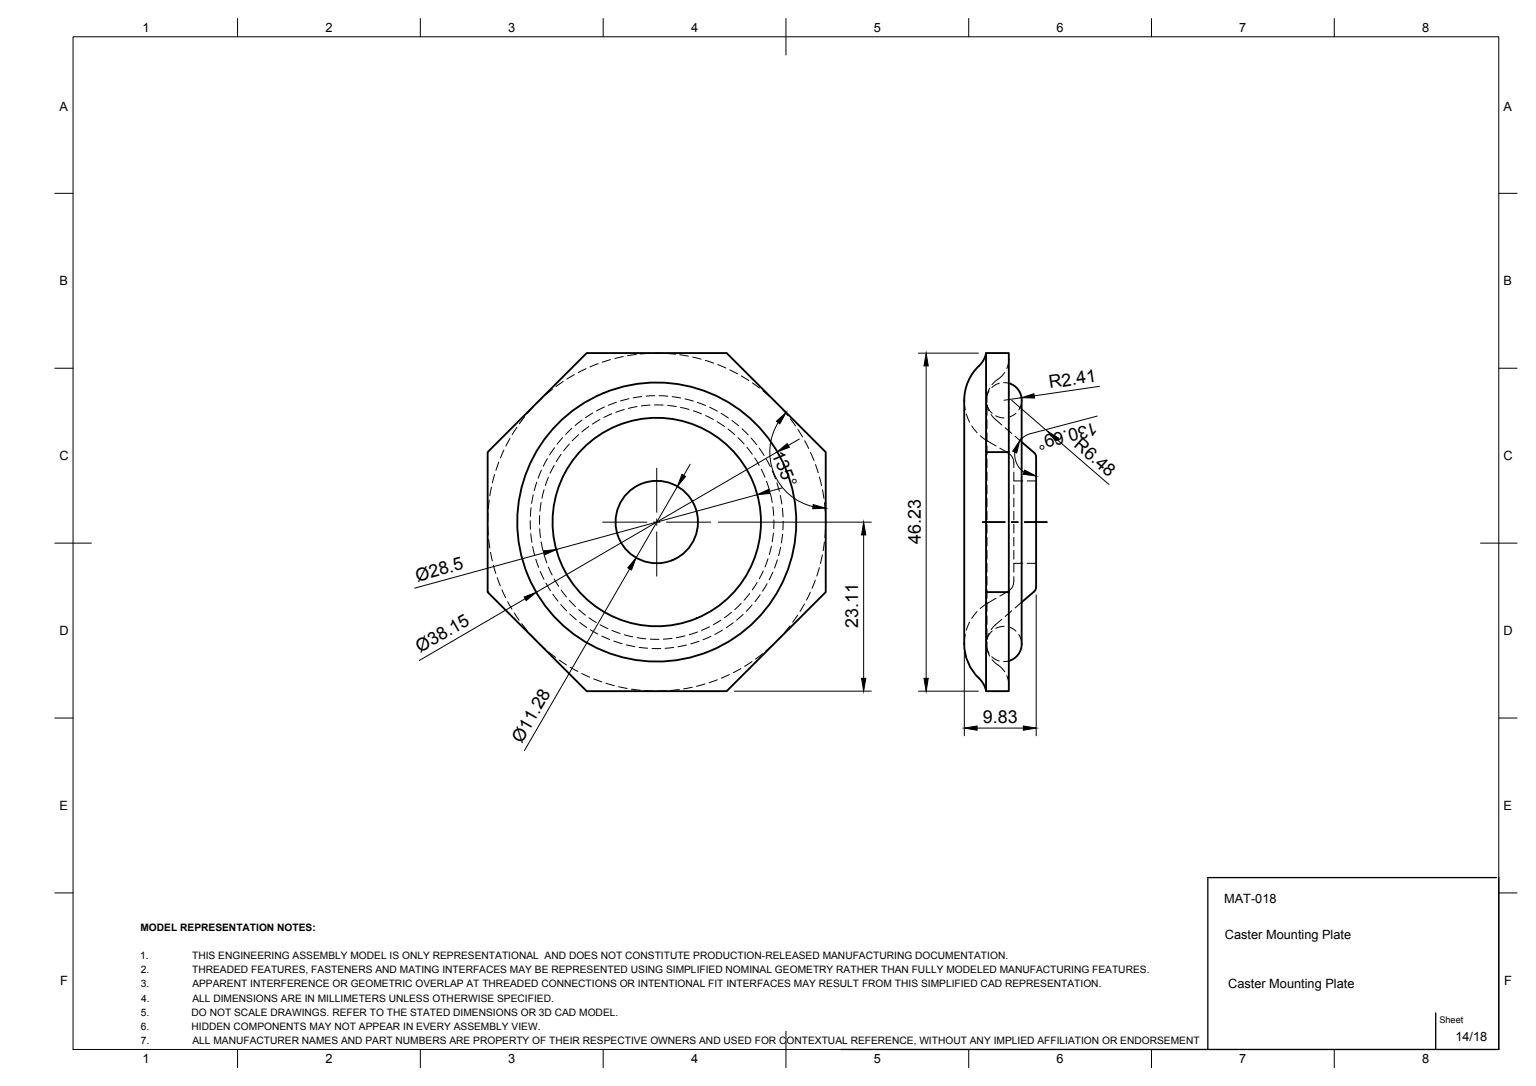
ISO-10303-21;
HEADER;
/* Generated by software containing ST-Developer
 * from STEP Tools, Inc. (www.steptools.com) 
 */

FILE_DESCRIPTION(
/* description */ ('STEP AP214'),
/* implementation_level */ '2;1');

FILE_NAME(
/* name */ 'Caster Mounting Plate.step',
/* time_stamp */ '2026-11-14T06:16:09-08:00',
/* author */ (''),
/* organization */ (''),
/* preprocessor_version */ 'ST-DEVELOPER v20.2',
/* originating_system */ 'Autodesk Translation Framework v15.17.0.0',
/* authorisation */ '');

FILE_SCHEMA (('AUTOMOTIVE_DESIGN { 1 0 10303 214 3 1 1 }'));
ENDSEC;

DATA;
#10=MECHANICAL_DESIGN_GEOMETRIC_PRESENTATION_REPRESENTATION('',(#358),#18006);
#141=CONICAL_SURFACE('',#10700,9.49667180024818,0.710179331162308);
#142=CONICAL_SURFACE('',#10715,11.0475234888716,0.521857699344453);
#252=TOROIDAL_SURFACE('',#10684,16.6624,2.413127);
#253=TOROIDAL_SURFACE('',#10688,16.6624,3.429);
#254=TOROIDAL_SURFACE('',#10695,8.89,0.8001);
#255=TOROIDAL_SURFACE('',#10701,16.6624,3.429);
#256=TOROIDAL_SURFACE('',#10704,22.296392545256,3.302);
#257=TOROIDAL_SURFACE('',#10707,23.7562339422346,3.302);
#258=TOROIDAL_SURFACE('',#10711,16.6624,6.477);
#259=TOROIDAL_SURFACE('',#10718,8.0899,1.6002);
#326=SHAPE_REPRESENTATION_RELATIONSHIP('SRR','None',#18084,#342);
#342=ADVANCED_BREP_SHAPE_REPRESENTATION('',(#374),#18001);
#358=STYLED_ITEM('',(#18172),#374);
#374=MANIFOLD_SOLID_BREP('Body1',#9567);
#482=FACE_BOUND('',#2048,.T.);
#483=FACE_BOUND('',#2050,.T.);
#484=FACE_BOUND('',#2052,.T.);
#485=FACE_BOUND('',#2054,.T.);
#813=PLANE('',#10721);
#814=PLANE('',#10722);
#815=PLANE('',#10723);
#816=PLANE('',#10724);
#817=PLANE('',#10725);
#818=PLANE('',#10726);
#819=PLANE('',#10727);
#820=PLANE('',#10728);
#821=PLANE('',#10729);
#822=PLANE('',#10730);
#823=PLANE('',#10731);
#824=PLANE('',#10732);
#1349=FACE_OUTER_BOUND('',#2028,.T.);
#1350=FACE_OUTER_BOUND('',#2029,.T.);
#1351=FACE_OUTER_BOUND('',#2030,.T.);
#1352=FACE_OUTER_BOUND('',#2031,.T.);
#1353=FACE_OUTER_BOUND('',#2032,.T.);
#1354=FACE_OUTER_BOUND('',#2033,.T.);
#1355=FACE_OUTER_BOUND('',#2034,.T.);
#1356=FACE_OUTER_BOUND('',#2035,.T.);
#1357=FACE_OUTER_BOUND('',#2036,.T.);
#1358=FACE_OUTER_BOUND('',#2037,.T.);
#1359=FACE_OUTER_BOUND('',#2038,.T.);
#1360=FACE_OUTER_BOUND('',#2039,.T.);
#1361=FACE_OUTER_BOUND('',#2040,.T.);
#1362=FACE_OUTER_BOUND('',#2041,.T.);
#1363=FACE_OUTER_BOUND('',#2042,.T.);
#1364=FACE_OUTER_BOUND('',#2043,.T.);
#1365=FACE_OUTER_BOUND('',#2044,.T.);
#1366=FACE_OUTER_BOUND('',#2045,.T.);
#1367=FACE_OUTER_BOUND('',#2046,.T.);
#1368=FACE_OUTER_BOUND('',#2047,.T.);
#1369=FACE_OUTER_BOUND('',#2049,.T.);
#1370=FACE_OUTER_BOUND('',#2051,.T.);
#1371=FACE_OUTER_BOUND('',#2053,.T.);
#2028=EDGE_LOOP('',(#8544,#8545,#8546,#8547));
#2029=EDGE_LOOP('',(#8548,#8549,#8550,#8551,#8552));
#2030=EDGE_LOOP('',(#8553,#8554,#8555,#8556));
#2031=EDGE_LOOP('',(#8557,#8558,#8559,#8560,#8561));
#2032=EDGE_LOOP('',(#8562,#8563,#8564,#8565,#8566,#8567));
#2033=EDGE_LOOP('',(#8568,#8569,#8570,#8571));
#2034=EDGE_LOOP('',(#8572,#8573,#8574,#8575));
#2035=EDGE_LOOP('',(#8576,#8577,#8578,#8579));
#2036=EDGE_LOOP('',(#8580,#8581,#8582,#8583,#8584));
#2037=EDGE_LOOP('',(#8585,#8586,#8587,#8588,#8589,#8590));
#2038=EDGE_LOOP('',(#8591,#8592,#8593,#8594,#8595));
#2039=EDGE_LOOP('',(#8596,#8597,#8598,#8599));
#2040=EDGE_LOOP('',(#8600,#8601,#8602,#8603));
#2041=EDGE_LOOP('',(#8604,#8605,#8606,#8607));
#2042=EDGE_LOOP('',(#8608,#8609,#8610,#8611));
#2043=EDGE_LOOP('',(#8612,#8613,#8614,#8615));
#2044=EDGE_LOOP('',(#8616,#8617,#8618,#8619));
#2045=EDGE_LOOP('',(#8620,#8621,#8622,#8623));
#2046=EDGE_LOOP('',(#8624,#8625,#8626,#8627));
#2047=EDGE_LOOP('',(#8628,#8629,#8630,#8631,#8632,#8633,#8634,#8635));
#2048=EDGE_LOOP('',(#8636));
#2049=EDGE_LOOP('',(#8637,#8638,#8639,#8640,#8641,#8642,#8643,#8644));
#2050=EDGE_LOOP('',(#8645));
#2051=EDGE_LOOP('',(#8646));
#2052=EDGE_LOOP('',(#8647));
#2053=EDGE_LOOP('',(#8648));
#2054=EDGE_LOOP('',(#8649));
#2792=LINE('',#17674,#3516);
#2793=LINE('',#17685,#3517);
#2794=LINE('',#17710,#3518);
#2795=LINE('',#17719,#3519);
#2796=LINE('',#17721,#3520);
#2797=LINE('',#17723,#3521);
#2798=LINE('',#17724,#3522);
#2799=LINE('',#17727,#3523);
#2800=LINE('',#17729,#3524);
#2801=LINE('',#17730,#3525);
#2802=LINE('',#17733,#3526);
#2803=LINE('',#17735,#3527);
#2804=LINE('',#17736,#3528);
#2805=LINE('',#17739,#3529);
#2806=LINE('',#17741,#3530);
#2807=LINE('',#17742,#3531);
#2808=LINE('',#17745,#3532);
#2809=LINE('',#17747,#3533);
#2810=LINE('',#17748,#3534);
#2811=LINE('',#17751,#3535);
#2812=LINE('',#17753,#3536);
#2813=LINE('',#17754,#3537);
#2814=LINE('',#17757,#3538);
#2815=LINE('',#17759,#3539);
#2816=LINE('',#17760,#3540);
#2817=LINE('',#17762,#3541);
#2818=LINE('',#17763,#3542);
#3516=VECTOR('',#13427,5.6388);
#3517=VECTOR('',#13442,9.49667180024818);
#3518=VECTOR('',#13475,11.0475234888716);
#3519=VECTOR('',#13486,1000.);
#3520=VECTOR('',#13487,1000.);
#3521=VECTOR('',#13488,1000.);
#3522=VECTOR('',#13489,1000.);
#3523=VECTOR('',#13492,1000.);
#3524=VECTOR('',#13493,1000.);
#3525=VECTOR('',#13494,1000.);
#3526=VECTOR('',#13497,1000.);
#3527=VECTOR('',#13498,1000.);
#3528=VECTOR('',#13499,1000.);
#3529=VECTOR('',#13502,1000.);
#3530=VECTOR('',#13503,1000.);
#3531=VECTOR('',#13504,1000.);
#3532=VECTOR('',#13507,1000.);
#3533=VECTOR('',#13508,1000.);
#3534=VECTOR('',#13509,1000.);
#3535=VECTOR('',#13512,1000.);
#3536=VECTOR('',#13513,1000.);
#3537=VECTOR('',#13514,1000.);
#3538=VECTOR('',#13517,1000.);
#3539=VECTOR('',#13518,1000.);
#3540=VECTOR('',#13519,1000.);
#3541=VECTOR('',#13522,1000.);
#3542=VECTOR('',#13523,1000.);
#3929=CIRCLE('',#10685,16.0314200400514);
#3930=CIRCLE('',#10686,2.413127);
#3931=CIRCLE('',#10687,17.2933799599486);
#3932=CIRCLE('',#10689,14.0623779989364);
#3933=CIRCLE('',#10690,14.0623779989364);
#3934=CIRCLE('',#10691,3.429);
#3935=CIRCLE('',#10693,5.6388);
#3936=CIRCLE('',#10694,5.6388);
#3937=CIRCLE('',#10696,8.89);
#3938=CIRCLE('',#10697,0.8001);
#3939=CIRCLE('',#10698,9.49667180024818);
#3940=CIRCLE('',#10699,9.49667180024818);
#3941=CIRCLE('',#10702,3.429);
#3942=CIRCLE('',#10703,19.5325471456964);
#3943=CIRCLE('',#10705,3.302);
#3944=CIRCLE('',#10706,22.296392545256);
#3945=CIRCLE('',#10708,23.1013);
#3946=CIRCLE('',#10709,3.302);
#3947=CIRCLE('',#10710,21.3609133903113);
#3948=CIRCLE('',#10712,6.477);
#3949=CIRCLE('',#10713,11.0475234888716);
#3950=CIRCLE('',#10714,11.0475234888716);
#3951=CIRCLE('',#10716,9.4771047851023);
#3952=CIRCLE('',#10717,9.4771047851023);
#3953=CIRCLE('',#10719,1.6002);
#3954=CIRCLE('',#10720,8.0899);
#4740=VERTEX_POINT('',#17659);
#4741=VERTEX_POINT('',#17661);
#4742=VERTEX_POINT('',#17665);
#4743=VERTEX_POINT('',#17666);
#4744=VERTEX_POINT('',#17671);
#4745=VERTEX_POINT('',#17673);
#4746=VERTEX_POINT('',#17677);
#4747=VERTEX_POINT('',#17679);
#4748=VERTEX_POINT('',#17681);
#4749=VERTEX_POINT('',#17687);
#4750=VERTEX_POINT('',#17691);
#4751=VERTEX_POINT('',#17695);
#4752=VERTEX_POINT('',#17697);
#4753=VERTEX_POINT('',#17701);
#4754=VERTEX_POINT('',#17703);
#4755=VERTEX_POINT('',#17707);
#4756=VERTEX_POINT('',#17708);
#4757=VERTEX_POINT('',#17713);
#4758=VERTEX_POINT('',#17717);
#4759=VERTEX_POINT('',#17718);
#4760=VERTEX_POINT('',#17720);
#4761=VERTEX_POINT('',#17722);
#4762=VERTEX_POINT('',#17726);
#4763=VERTEX_POINT('',#17728);
#4764=VERTEX_POINT('',#17732);
#4765=VERTEX_POINT('',#17734);
#4766=VERTEX_POINT('',#17738);
#4767=VERTEX_POINT('',#17740);
#4768=VERTEX_POINT('',#17744);
#4769=VERTEX_POINT('',#17746);
#4770=VERTEX_POINT('',#17750);
#4771=VERTEX_POINT('',#17752);
#4772=VERTEX_POINT('',#17756);
#4773=VERTEX_POINT('',#17758);
#6020=EDGE_CURVE('',#4740,#4740,#3929,.T.);
#6021=EDGE_CURVE('',#4740,#4741,#3930,.T.);
#6022=EDGE_CURVE('',#4741,#4741,#3931,.T.);
#6023=EDGE_CURVE('',#4742,#4743,#3932,.T.);
#6024=EDGE_CURVE('',#4743,#4742,#3933,.T.);
#6025=EDGE_CURVE('',#4743,#4740,#3934,.T.);
#6026=EDGE_CURVE('',#4744,#4744,#3935,.T.);
#6027=EDGE_CURVE('',#4744,#4745,#2792,.T.);
#6028=EDGE_CURVE('',#4745,#4745,#3936,.T.);
#6029=EDGE_CURVE('',#4746,#4746,#3937,.T.);
#6030=EDGE_CURVE('',#4746,#4747,#3938,.T.);
#6031=EDGE_CURVE('',#4747,#4748,#3939,.T.);
#6032=EDGE_CURVE('',#4748,#4747,#3940,.T.);
#6033=EDGE_CURVE('',#4742,#4748,#2793,.T.);
#6034=EDGE_CURVE('',#4741,#4749,#3941,.T.);
#6035=EDGE_CURVE('',#4749,#4749,#3942,.T.);
#6036=EDGE_CURVE('',#4749,#4750,#3943,.T.);
#6037=EDGE_CURVE('',#4750,#4750,#3944,.T.);
#6038=EDGE_CURVE('',#4751,#4751,#3945,.T.);
#6039=EDGE_CURVE('',#4751,#4752,#3946,.T.);
#6040=EDGE_CURVE('',#4752,#4752,#3947,.T.);
#6041=EDGE_CURVE('',#4752,#4753,#3948,.T.);
#6042=EDGE_CURVE('',#4753,#4754,#3949,.T.);
#6043=EDGE_CURVE('',#4754,#4753,#3950,.T.);
#6044=EDGE_CURVE('',#4755,#4756,#3951,.T.);
#6045=EDGE_CURVE('',#4756,#4754,#2794,.T.);
#6046=EDGE_CURVE('',#4756,#4755,#3952,.T.);
#6047=EDGE_CURVE('',#4755,#4757,#3953,.T.);
#6048=EDGE_CURVE('',#4757,#4757,#3954,.T.);
#6049=EDGE_CURVE('',#4758,#4759,#2795,.T.);
#6050=EDGE_CURVE('',#4760,#4759,#2796,.T.);
#6051=EDGE_CURVE('',#4760,#4761,#2797,.T.);
#6052=EDGE_CURVE('',#4761,#4758,#2798,.T.);
#6053=EDGE_CURVE('',#4759,#4762,#2799,.T.);
#6054=EDGE_CURVE('',#4763,#4762,#2800,.T.);
#6055=EDGE_CURVE('',#4763,#4760,#2801,.T.);
#6056=EDGE_CURVE('',#4762,#4764,#2802,.T.);
#6057=EDGE_CURVE('',#4765,#4764,#2803,.T.);
#6058=EDGE_CURVE('',#4765,#4763,#2804,.T.);
#6059=EDGE_CURVE('',#4764,#4766,#2805,.T.);
#6060=EDGE_CURVE('',#4767,#4766,#2806,.T.);
#6061=EDGE_CURVE('',#4767,#4765,#2807,.T.);
#6062=EDGE_CURVE('',#4766,#4768,#2808,.T.);
#6063=EDGE_CURVE('',#4769,#4768,#2809,.T.);
#6064=EDGE_CURVE('',#4769,#4767,#2810,.T.);
#6065=EDGE_CURVE('',#4768,#4770,#2811,.T.);
#6066=EDGE_CURVE('',#4771,#4770,#2812,.T.);
#6067=EDGE_CURVE('',#4771,#4769,#2813,.T.);
#6068=EDGE_CURVE('',#4770,#4772,#2814,.T.);
#6069=EDGE_CURVE('',#4773,#4772,#2815,.T.);
#6070=EDGE_CURVE('',#4773,#4771,#2816,.T.);
#6071=EDGE_CURVE('',#4772,#4758,#2817,.T.);
#6072=EDGE_CURVE('',#4761,#4773,#2818,.T.);
#8544=ORIENTED_EDGE('',*,*,#6020,.F.);
#8545=ORIENTED_EDGE('',*,*,#6021,.T.);
#8546=ORIENTED_EDGE('',*,*,#6022,.F.);
#8547=ORIENTED_EDGE('',*,*,#6021,.F.);
#8548=ORIENTED_EDGE('',*,*,#6023,.F.);
#8549=ORIENTED_EDGE('',*,*,#6024,.F.);
#8550=ORIENTED_EDGE('',*,*,#6025,.T.);
#8551=ORIENTED_EDGE('',*,*,#6020,.T.);
#8552=ORIENTED_EDGE('',*,*,#6025,.F.);
#8553=ORIENTED_EDGE('',*,*,#6026,.F.);
#8554=ORIENTED_EDGE('',*,*,#6027,.T.);
#8555=ORIENTED_EDGE('',*,*,#6028,.T.);
#8556=ORIENTED_EDGE('',*,*,#6027,.F.);
#8557=ORIENTED_EDGE('',*,*,#6029,.F.);
#8558=ORIENTED_EDGE('',*,*,#6030,.T.);
#8559=ORIENTED_EDGE('',*,*,#6031,.T.);
#8560=ORIENTED_EDGE('',*,*,#6032,.T.);
#8561=ORIENTED_EDGE('',*,*,#6030,.F.);
#8562=ORIENTED_EDGE('',*,*,#6023,.T.);
#8563=ORIENTED_EDGE('',*,*,#6024,.T.);
#8564=ORIENTED_EDGE('',*,*,#6033,.T.);
#8565=ORIENTED_EDGE('',*,*,#6031,.F.);
#8566=ORIENTED_EDGE('',*,*,#6032,.F.);
#8567=ORIENTED_EDGE('',*,*,#6033,.F.);
#8568=ORIENTED_EDGE('',*,*,#6022,.T.);
#8569=ORIENTED_EDGE('',*,*,#6034,.T.);
#8570=ORIENTED_EDGE('',*,*,#6035,.T.);
#8571=ORIENTED_EDGE('',*,*,#6034,.F.);
#8572=ORIENTED_EDGE('',*,*,#6035,.F.);
#8573=ORIENTED_EDGE('',*,*,#6036,.T.);
#8574=ORIENTED_EDGE('',*,*,#6037,.T.);
#8575=ORIENTED_EDGE('',*,*,#6036,.F.);
#8576=ORIENTED_EDGE('',*,*,#6038,.F.);
#8577=ORIENTED_EDGE('',*,*,#6039,.T.);
#8578=ORIENTED_EDGE('',*,*,#6040,.T.);
#8579=ORIENTED_EDGE('',*,*,#6039,.F.);
#8580=ORIENTED_EDGE('',*,*,#6040,.F.);
#8581=ORIENTED_EDGE('',*,*,#6041,.T.);
#8582=ORIENTED_EDGE('',*,*,#6042,.T.);
#8583=ORIENTED_EDGE('',*,*,#6043,.T.);
#8584=ORIENTED_EDGE('',*,*,#6041,.F.);
#8585=ORIENTED_EDGE('',*,*,#6044,.T.);
#8586=ORIENTED_EDGE('',*,*,#6045,.T.);
#8587=ORIENTED_EDGE('',*,*,#6042,.F.);
#8588=ORIENTED_EDGE('',*,*,#6043,.F.);
#8589=ORIENTED_EDGE('',*,*,#6045,.F.);
#8590=ORIENTED_EDGE('',*,*,#6046,.T.);
#8591=ORIENTED_EDGE('',*,*,#6044,.F.);
#8592=ORIENTED_EDGE('',*,*,#6047,.T.);
#8593=ORIENTED_EDGE('',*,*,#6048,.T.);
#8594=ORIENTED_EDGE('',*,*,#6047,.F.);
#8595=ORIENTED_EDGE('',*,*,#6046,.F.);
#8596=ORIENTED_EDGE('',*,*,#6049,.T.);
#8597=ORIENTED_EDGE('',*,*,#6050,.F.);
#8598=ORIENTED_EDGE('',*,*,#6051,.T.);
#8599=ORIENTED_EDGE('',*,*,#6052,.T.);
#8600=ORIENTED_EDGE('',*,*,#6053,.T.);
#8601=ORIENTED_EDGE('',*,*,#6054,.F.);
#8602=ORIENTED_EDGE('',*,*,#6055,.T.);
#8603=ORIENTED_EDGE('',*,*,#6050,.T.);
#8604=ORIENTED_EDGE('',*,*,#6056,.T.);
#8605=ORIENTED_EDGE('',*,*,#6057,.F.);
#8606=ORIENTED_EDGE('',*,*,#6058,.T.);
#8607=ORIENTED_EDGE('',*,*,#6054,.T.);
#8608=ORIENTED_EDGE('',*,*,#6059,.T.);
#8609=ORIENTED_EDGE('',*,*,#6060,.F.);
#8610=ORIENTED_EDGE('',*,*,#6061,.T.);
#8611=ORIENTED_EDGE('',*,*,#6057,.T.);
#8612=ORIENTED_EDGE('',*,*,#6062,.T.);
#8613=ORIENTED_EDGE('',*,*,#6063,.F.);
#8614=ORIENTED_EDGE('',*,*,#6064,.T.);
#8615=ORIENTED_EDGE('',*,*,#6060,.T.);
#8616=ORIENTED_EDGE('',*,*,#6065,.T.);
#8617=ORIENTED_EDGE('',*,*,#6066,.F.);
#8618=ORIENTED_EDGE('',*,*,#6067,.T.);
#8619=ORIENTED_EDGE('',*,*,#6063,.T.);
#8620=ORIENTED_EDGE('',*,*,#6068,.T.);
#8621=ORIENTED_EDGE('',*,*,#6069,.F.);
#8622=ORIENTED_EDGE('',*,*,#6070,.T.);
#8623=ORIENTED_EDGE('',*,*,#6066,.T.);
#8624=ORIENTED_EDGE('',*,*,#6071,.T.);
#8625=ORIENTED_EDGE('',*,*,#6052,.F.);
#8626=ORIENTED_EDGE('',*,*,#6072,.T.);
#8627=ORIENTED_EDGE('',*,*,#6069,.T.);
#8628=ORIENTED_EDGE('',*,*,#6072,.F.);
#8629=ORIENTED_EDGE('',*,*,#6051,.F.);
#8630=ORIENTED_EDGE('',*,*,#6055,.F.);
#8631=ORIENTED_EDGE('',*,*,#6058,.F.);
#8632=ORIENTED_EDGE('',*,*,#6061,.F.);
#8633=ORIENTED_EDGE('',*,*,#6064,.F.);
#8634=ORIENTED_EDGE('',*,*,#6067,.F.);
#8635=ORIENTED_EDGE('',*,*,#6070,.F.);
#8636=ORIENTED_EDGE('',*,*,#6038,.T.);
#8637=ORIENTED_EDGE('',*,*,#6071,.F.);
#8638=ORIENTED_EDGE('',*,*,#6068,.F.);
#8639=ORIENTED_EDGE('',*,*,#6065,.F.);
#8640=ORIENTED_EDGE('',*,*,#6062,.F.);
#8641=ORIENTED_EDGE('',*,*,#6059,.F.);
#8642=ORIENTED_EDGE('',*,*,#6056,.F.);
#8643=ORIENTED_EDGE('',*,*,#6053,.F.);
#8644=ORIENTED_EDGE('',*,*,#6049,.F.);
#8645=ORIENTED_EDGE('',*,*,#6037,.F.);
#8646=ORIENTED_EDGE('',*,*,#6029,.T.);
#8647=ORIENTED_EDGE('',*,*,#6028,.F.);
#8648=ORIENTED_EDGE('',*,*,#6048,.F.);
#8649=ORIENTED_EDGE('',*,*,#6026,.T.);
#8968=CYLINDRICAL_SURFACE('',#10692,5.6388);
#9488=ADVANCED_FACE('',(#1349),#252,.T.);
#9489=ADVANCED_FACE('',(#1350),#253,.F.);
#9490=ADVANCED_FACE('',(#1351),#8968,.F.);
#9491=ADVANCED_FACE('',(#1352),#254,.T.);
#9492=ADVANCED_FACE('',(#1353),#141,.T.);
#9493=ADVANCED_FACE('',(#1354),#255,.F.);
#9494=ADVANCED_FACE('',(#1355),#256,.T.);
#9495=ADVANCED_FACE('',(#1356),#257,.F.);
#9496=ADVANCED_FACE('',(#1357),#258,.T.);
#9497=ADVANCED_FACE('',(#1358),#142,.F.);
#9498=ADVANCED_FACE('',(#1359),#259,.F.);
#9499=ADVANCED_FACE('',(#1360),#813,.F.);
#9500=ADVANCED_FACE('',(#1361),#814,.F.);
#9501=ADVANCED_FACE('',(#1362),#815,.F.);
#9502=ADVANCED_FACE('',(#1363),#816,.F.);
#9503=ADVANCED_FACE('',(#1364),#817,.F.);
#9504=ADVANCED_FACE('',(#1365),#818,.F.);
#9505=ADVANCED_FACE('',(#1366),#819,.F.);
#9506=ADVANCED_FACE('',(#1367),#820,.F.);
#9507=ADVANCED_FACE('',(#1368,#482),#821,.T.);
#9508=ADVANCED_FACE('',(#1369,#483),#822,.T.);
#9509=ADVANCED_FACE('',(#1370,#484),#823,.T.);
#9510=ADVANCED_FACE('',(#1371,#485),#824,.T.);
#9567=CLOSED_SHELL('',(#9488,#9489,#9490,#9491,#9492,#9493,#9494,#9495,
#9496,#9497,#9498,#9499,#9500,#9501,#9502,#9503,#9504,#9505,#9506,#9507,
#9508,#9509,#9510));
#10683=AXIS2_PLACEMENT_3D('',#17657,#13405,#13406);
#10684=AXIS2_PLACEMENT_3D('',#17658,#13407,#13408);
#10685=AXIS2_PLACEMENT_3D('',#17660,#13409,#13410);
#10686=AXIS2_PLACEMENT_3D('',#17662,#13411,#13412);
#10687=AXIS2_PLACEMENT_3D('',#17663,#13413,#13414);
#10688=AXIS2_PLACEMENT_3D('',#17664,#13415,#13416);
#10689=AXIS2_PLACEMENT_3D('',#17667,#13417,#13418);
#10690=AXIS2_PLACEMENT_3D('',#17668,#13419,#13420);
#10691=AXIS2_PLACEMENT_3D('',#17669,#13421,#13422);
#10692=AXIS2_PLACEMENT_3D('',#17670,#13423,#13424);
#10693=AXIS2_PLACEMENT_3D('',#17672,#13425,#13426);
#10694=AXIS2_PLACEMENT_3D('',#17675,#13428,#13429);
#10695=AXIS2_PLACEMENT_3D('',#17676,#13430,#13431);
#10696=AXIS2_PLACEMENT_3D('',#17678,#13432,#13433);
#10697=AXIS2_PLACEMENT_3D('',#17680,#13434,#13435);
#10698=AXIS2_PLACEMENT_3D('',#17682,#13436,#13437);
#10699=AXIS2_PLACEMENT_3D('',#17683,#13438,#13439);
#10700=AXIS2_PLACEMENT_3D('',#17684,#13440,#13441);
#10701=AXIS2_PLACEMENT_3D('',#17686,#13443,#13444);
#10702=AXIS2_PLACEMENT_3D('',#17688,#13445,#13446);
#10703=AXIS2_PLACEMENT_3D('',#17689,#13447,#13448);
#10704=AXIS2_PLACEMENT_3D('',#17690,#13449,#13450);
#10705=AXIS2_PLACEMENT_3D('',#17692,#13451,#13452);
#10706=AXIS2_PLACEMENT_3D('',#17693,#13453,#13454);
#10707=AXIS2_PLACEMENT_3D('',#17694,#13455,#13456);
#10708=AXIS2_PLACEMENT_3D('',#17696,#13457,#13458);
#10709=AXIS2_PLACEMENT_3D('',#17698,#13459,#13460);
#10710=AXIS2_PLACEMENT_3D('',#17699,#13461,#13462);
#10711=AXIS2_PLACEMENT_3D('',#17700,#13463,#13464);
#10712=AXIS2_PLACEMENT_3D('',#17702,#13465,#13466);
#10713=AXIS2_PLACEMENT_3D('',#17704,#13467,#13468);
#10714=AXIS2_PLACEMENT_3D('',#17705,#13469,#13470);
#10715=AXIS2_PLACEMENT_3D('',#17706,#13471,#13472);
#10716=AXIS2_PLACEMENT_3D('',#17709,#13473,#13474);
#10717=AXIS2_PLACEMENT_3D('',#17711,#13476,#13477);
#10718=AXIS2_PLACEMENT_3D('',#17712,#13478,#13479);
#10719=AXIS2_PLACEMENT_3D('',#17714,#13480,#13481);
#10720=AXIS2_PLACEMENT_3D('',#17715,#13482,#13483);
#10721=AXIS2_PLACEMENT_3D('',#17716,#13484,#13485);
#10722=AXIS2_PLACEMENT_3D('',#17725,#13490,#13491);
#10723=AXIS2_PLACEMENT_3D('',#17731,#13495,#13496);
#10724=AXIS2_PLACEMENT_3D('',#17737,#13500,#13501);
#10725=AXIS2_PLACEMENT_3D('',#17743,#13505,#13506);
#10726=AXIS2_PLACEMENT_3D('',#17749,#13510,#13511);
#10727=AXIS2_PLACEMENT_3D('',#17755,#13515,#13516);
#10728=AXIS2_PLACEMENT_3D('',#17761,#13520,#13521);
#10729=AXIS2_PLACEMENT_3D('',#17764,#13524,#13525);
#10730=AXIS2_PLACEMENT_3D('',#17765,#13526,#13527);
#10731=AXIS2_PLACEMENT_3D('',#17766,#13528,#13529);
#10732=AXIS2_PLACEMENT_3D('',#17767,#13530,#13531);
#13405=DIRECTION('axis',(0.,0.,1.));
#13406=DIRECTION('refdir',(1.,0.,0.));
#13407=DIRECTION('center_axis',(0.,-1.,0.));
#13408=DIRECTION('ref_axis',(0.,0.,-1.));
#13409=DIRECTION('center_axis',(0.,-1.,0.));
#13410=DIRECTION('ref_axis',(0.,0.,-1.));
#13411=DIRECTION('center_axis',(-1.,0.,-1.22464679914735E-16));
#13412=DIRECTION('ref_axis',(-1.22464679914735E-16,0.,1.));
#13413=DIRECTION('center_axis',(0.,1.,0.));
#13414=DIRECTION('ref_axis',(0.,0.,1.));
#13415=DIRECTION('center_axis',(0.,-1.,0.));
#13416=DIRECTION('ref_axis',(0.,0.,-1.));
#13417=DIRECTION('center_axis',(0.,-1.,0.));
#13418=DIRECTION('ref_axis',(0.,0.,-1.));
#13419=DIRECTION('center_axis',(0.,-1.,0.));
#13420=DIRECTION('ref_axis',(0.,0.,-1.));
#13421=DIRECTION('center_axis',(1.,0.,1.22464679914735E-16));
#13422=DIRECTION('ref_axis',(-1.22464679914735E-16,0.,1.));
#13423=DIRECTION('center_axis',(0.,-1.,0.));
#13424=DIRECTION('ref_axis',(0.,0.,-1.));
#13425=DIRECTION('center_axis',(0.,-1.,0.));
#13426=DIRECTION('ref_axis',(0.,0.,-1.));
#13427=DIRECTION('',(0.,-1.,0.));
#13428=DIRECTION('center_axis',(0.,-1.,0.));
#13429=DIRECTION('ref_axis',(0.,0.,-1.));
#13430=DIRECTION('center_axis',(0.,-1.,0.));
#13431=DIRECTION('ref_axis',(0.,0.,-1.));
#13432=DIRECTION('center_axis',(0.,-1.,0.));
#13433=DIRECTION('ref_axis',(0.,0.,-1.));
#13434=DIRECTION('center_axis',(-1.,0.,-1.22464679914735E-16));
#13435=DIRECTION('ref_axis',(-1.22464679914735E-16,0.,1.));
#13436=DIRECTION('center_axis',(0.,-1.,0.));
#13437=DIRECTION('ref_axis',(0.,0.,-1.));
#13438=DIRECTION('center_axis',(0.,-1.,0.));
#13439=DIRECTION('ref_axis',(0.,0.,-1.));
#13440=DIRECTION('center_axis',(0.,1.,0.));
#13441=DIRECTION('ref_axis',(0.,0.,1.));
#13442=DIRECTION('',(7.98432677834137E-17,-0.758244969689014,0.651969758456101));
#13443=DIRECTION('center_axis',(0.,-1.,0.));
#13444=DIRECTION('ref_axis',(0.,0.,-1.));
#13445=DIRECTION('center_axis',(1.,0.,1.22464679914735E-16));
#13446=DIRECTION('ref_axis',(-1.22464679914735E-16,0.,1.));
#13447=DIRECTION('center_axis',(0.,-1.,0.));
#13448=DIRECTION('ref_axis',(0.,0.,-1.));
#13449=DIRECTION('center_axis',(0.,-1.,0.));
#13450=DIRECTION('ref_axis',(0.,0.,-1.));
#13451=DIRECTION('center_axis',(-1.,0.,-1.22464679914735E-16));
#13452=DIRECTION('ref_axis',(-1.22464679914735E-16,0.,1.));
#13453=DIRECTION('center_axis',(0.,-1.,0.));
#13454=DIRECTION('ref_axis',(0.,0.,-1.));
#13455=DIRECTION('center_axis',(0.,-1.,0.));
#13456=DIRECTION('ref_axis',(0.,0.,-1.));
#13457=DIRECTION('center_axis',(0.,-1.,0.));
#13458=DIRECTION('ref_axis',(0.,0.,-1.));
#13459=DIRECTION('center_axis',(1.,0.,1.22464679914735E-16));
#13460=DIRECTION('ref_axis',(-1.22464679914735E-16,0.,1.));
#13461=DIRECTION('center_axis',(0.,-1.,0.));
#13462=DIRECTION('ref_axis',(0.,0.,-1.));
#13463=DIRECTION('center_axis',(0.,-1.,0.));
#13464=DIRECTION('ref_axis',(0.,0.,-1.));
#13465=DIRECTION('center_axis',(-1.,0.,-1.22464679914735E-16));
#13466=DIRECTION('ref_axis',(-1.22464679914735E-16,0.,1.));
#13467=DIRECTION('center_axis',(0.,-1.,0.));
#13468=DIRECTION('ref_axis',(0.,0.,-1.));
#13469=DIRECTION('center_axis',(0.,-1.,0.));
#13470=DIRECTION('ref_axis',(0.,0.,-1.));
#13471=DIRECTION('center_axis',(0.,1.,0.));
#13472=DIRECTION('ref_axis',(0.,0.,1.));
#13473=DIRECTION('center_axis',(0.,-1.,0.));
#13474=DIRECTION('ref_axis',(0.,0.,-1.));
#13475=DIRECTION('',(-6.10475930061065E-17,0.866894628860328,-0.49849142665959));
#13476=DIRECTION('center_axis',(0.,-1.,0.));
#13477=DIRECTION('ref_axis',(0.,0.,-1.));
#13478=DIRECTION('center_axis',(0.,-1.,0.));
#13479=DIRECTION('ref_axis',(0.,0.,-1.));
#13480=DIRECTION('center_axis',(1.,0.,1.22464679914735E-16));
#13481=DIRECTION('ref_axis',(-1.22464679914735E-16,0.,1.));
#13482=DIRECTION('center_axis',(0.,-1.,0.));
#13483=DIRECTION('ref_axis',(0.,0.,-1.));
#13484=DIRECTION('center_axis',(0.923879532511287,0.,-0.38268343236509));
#13485=DIRECTION('ref_axis',(0.,-1.,0.));
#13486=DIRECTION('',(0.38268343236509,0.,0.923879532511287));
#13487=DIRECTION('',(0.,-1.,0.));
#13488=DIRECTION('',(-0.38268343236509,0.,-0.923879532511287));
#13489=DIRECTION('',(0.,-1.,0.));
#13490=DIRECTION('center_axis',(0.38268343236509,0.,-0.923879532511287));
#13491=DIRECTION('ref_axis',(0.,-1.,0.));
#13492=DIRECTION('',(0.923879532511287,0.,0.38268343236509));
#13493=DIRECTION('',(0.,-1.,0.));
#13494=DIRECTION('',(-0.923879532511287,0.,-0.38268343236509));
#13495=DIRECTION('center_axis',(-0.38268343236509,0.,-0.923879532511287));
#13496=DIRECTION('ref_axis',(-0.923879532511287,0.,0.38268343236509));
#13497=DIRECTION('',(0.923879532511287,0.,-0.38268343236509));
#13498=DIRECTION('',(0.,-1.,0.));
#13499=DIRECTION('',(-0.923879532511287,0.,0.38268343236509));
#13500=DIRECTION('center_axis',(-0.923879532511287,0.,-0.38268343236509));
#13501=DIRECTION('ref_axis',(-0.38268343236509,0.,0.923879532511287));
#13502=DIRECTION('',(0.38268343236509,0.,-0.923879532511287));
#13503=DIRECTION('',(0.,-1.,0.));
#13504=DIRECTION('',(-0.38268343236509,0.,0.923879532511287));
#13505=DIRECTION('center_axis',(-0.923879532511287,0.,0.38268343236509));
#13506=DIRECTION('ref_axis',(0.,1.,0.));
#13507=DIRECTION('',(-0.38268343236509,0.,-0.923879532511287));
#13508=DIRECTION('',(0.,-1.,0.));
#13509=DIRECTION('',(0.38268343236509,0.,0.923879532511287));
#13510=DIRECTION('center_axis',(-0.38268343236509,0.,0.923879532511287));
#13511=DIRECTION('ref_axis',(0.,1.,0.));
#13512=DIRECTION('',(-0.923879532511287,0.,-0.38268343236509));
#13513=DIRECTION('',(0.,-1.,0.));
#13514=DIRECTION('',(0.923879532511287,0.,0.38268343236509));
#13515=DIRECTION('center_axis',(0.38268343236509,0.,0.923879532511287));
#13516=DIRECTION('ref_axis',(0.,-1.,0.));
#13517=DIRECTION('',(-0.923879532511287,0.,0.38268343236509));
#13518=DIRECTION('',(0.,-1.,0.));
#13519=DIRECTION('',(0.923879532511287,0.,-0.38268343236509));
#13520=DIRECTION('center_axis',(0.923879532511287,0.,0.38268343236509));
#13521=DIRECTION('ref_axis',(0.,-1.,0.));
#13522=DIRECTION('',(-0.38268343236509,0.,0.923879532511287));
#13523=DIRECTION('',(0.38268343236509,0.,-0.923879532511287));
#13524=DIRECTION('center_axis',(0.,1.,0.));
#13525=DIRECTION('ref_axis',(1.,0.,0.));
#13526=DIRECTION('center_axis',(0.,-1.,0.));
#13527=DIRECTION('ref_axis',(0.,0.,-1.));
#13528=DIRECTION('center_axis',(0.,-1.,0.));
#13529=DIRECTION('ref_axis',(0.,0.,-1.));
#13530=DIRECTION('center_axis',(0.,1.,0.));
#13531=DIRECTION('ref_axis',(1.,0.,0.));
#17657=CARTESIAN_POINT('',(0.,0.,0.));
#17658=CARTESIAN_POINT('Origin',(0.,4.394073,0.));
#17659=CARTESIAN_POINT('',(-1.96328272378357E-15,6.72324585925114,16.0314200400514));
#17660=CARTESIAN_POINT('Origin',(0.,6.72324585925114,0.));
#17661=CARTESIAN_POINT('',(-2.117828241439E-15,6.72324585925114,17.2933799599486));
#17662=CARTESIAN_POINT('Origin',(-2.04055548261129E-15,4.394073,16.6624));
#17663=CARTESIAN_POINT('Origin',(0.,6.72324585925114,0.));
#17664=CARTESIAN_POINT('Origin',(0.,3.3528,0.));
#17665=CARTESIAN_POINT('',(1.72214462047976E-15,5.58840430174598,-14.0623779989364));
#17666=CARTESIAN_POINT('',(-1.72214462047976E-15,5.58840430174598,14.0623779989364));
#17667=CARTESIAN_POINT('Origin',(0.,5.58840430174598,0.));
#17668=CARTESIAN_POINT('Origin',(0.,5.58840430174598,0.));
#17669=CARTESIAN_POINT('Origin',(-2.04055548261129E-15,3.3528,16.6624));
#17670=CARTESIAN_POINT('Origin',(0.,0.,0.));
#17671=CARTESIAN_POINT('',(-6.9055383710321E-16,3.048,5.6388));
#17672=CARTESIAN_POINT('Origin',(0.,3.048,0.));
#17673=CARTESIAN_POINT('',(-6.9055383710321E-16,0.,5.6388));
#17674=CARTESIAN_POINT('',(-6.9055383710321E-16,0.,5.6388));
#17675=CARTESIAN_POINT('Origin',(0.,0.,0.));
#17676=CARTESIAN_POINT('Origin',(0.,0.800099999999998,0.));
#17677=CARTESIAN_POINT('',(-1.088711004442E-15,0.,8.89));
#17678=CARTESIAN_POINT('Origin',(0.,0.,0.));
#17679=CARTESIAN_POINT('',(-1.16300687227269E-15,0.278458996259272,9.49667180024818));
#17680=CARTESIAN_POINT('Origin',(-1.088711004442E-15,0.800099999999998,
8.89));
#17681=CARTESIAN_POINT('',(1.44257574637622E-15,0.278458996259272,-9.49667180024818));
#17682=CARTESIAN_POINT('Origin',(0.,0.278458996259272,0.));
#17683=CARTESIAN_POINT('Origin',(0.,0.278458996259272,0.));
#17684=CARTESIAN_POINT('Origin',(0.,0.278458996259272,0.));
#17685=CARTESIAN_POINT('',(-1.16300687227269E-15,0.278458996259272,-9.49667180024818));
#17686=CARTESIAN_POINT('Origin',(0.,3.3528,0.));
#17687=CARTESIAN_POINT('',(-2.39204713411719E-15,5.22904528301887,19.5325471456964));
#17688=CARTESIAN_POINT('Origin',(-2.04055548261129E-15,3.3528,16.6624));
#17689=CARTESIAN_POINT('Origin',(0.,5.22904528301887,0.));
#17690=CARTESIAN_POINT('Origin',(0.,7.0358,0.));
#17691=CARTESIAN_POINT('',(-2.73052057630807E-15,3.7338,22.296392545256));
#17692=CARTESIAN_POINT('Origin',(-2.73052057630807E-15,7.0358,22.296392545256));
#17693=CARTESIAN_POINT('Origin',(0.,3.7338,0.));
#17694=CARTESIAN_POINT('Origin',(0.,10.0838,0.));
#17695=CARTESIAN_POINT('',(-2.82909331011428E-15,6.84740300159127,23.1013));
#17696=CARTESIAN_POINT('Origin',(0.,6.84740300159127,0.));
#17697=CARTESIAN_POINT('',(-2.61595742103085E-15,7.81099480519482,21.3609133903113));
#17698=CARTESIAN_POINT('Origin',(-2.90929958571533E-15,10.0838,23.7562339422346));
#17699=CARTESIAN_POINT('Origin',(0.,7.81099480519482,0.));
#17700=CARTESIAN_POINT('Origin',(0.,3.3528,0.));
#17701=CARTESIAN_POINT('',(-1.35293142791519E-15,6.58152897047418,11.0475234888716));
#17702=CARTESIAN_POINT('Origin',(-2.04055548261129E-15,3.3528,16.6624));
#17703=CARTESIAN_POINT('',(1.35293142791519E-15,6.58152897047418,-11.0475234888716));
#17704=CARTESIAN_POINT('Origin',(0.,6.58152897047418,0.));
#17705=CARTESIAN_POINT('Origin',(0.,6.58152897047418,0.));
#17706=CARTESIAN_POINT('Origin',(0.,6.58152897047418,0.));
#17707=CARTESIAN_POINT('',(1.16061060402596E-15,3.85051401905933,9.4771047851023));
#17708=CARTESIAN_POINT('',(-1.16061060402596E-15,3.85051401905934,-9.47710478510228));
#17709=CARTESIAN_POINT('Origin',(0.,3.85051401905933,0.));
#17710=CARTESIAN_POINT('',(-1.35293142791519E-15,6.58152897047418,-11.0475234888716));
#17711=CARTESIAN_POINT('Origin',(0.,3.85051401905933,0.));
#17712=CARTESIAN_POINT('Origin',(0.,4.6482,0.));
#17713=CARTESIAN_POINT('',(-9.90727014042217E-16,3.048,8.0899));
#17714=CARTESIAN_POINT('Origin',(-9.90727014042217E-16,4.6482,8.0899));
#17715=CARTESIAN_POINT('Origin',(0.,3.048,0.));
#17716=CARTESIAN_POINT('Origin',(-25.019,25.4,-1.94289029309402E-13));
#17717=CARTESIAN_POINT('',(-25.019,3.7338,-1.94289029309402E-13));
#17718=CARTESIAN_POINT('',(-17.6911045585062,3.7338,17.6911045585061));
#17719=CARTESIAN_POINT('',(-18.089821188999,3.7338,16.7285174616265));
#17720=CARTESIAN_POINT('',(-17.6911045585062,6.84740300159127,17.6911045585061));
#17721=CARTESIAN_POINT('',(-17.6911045585062,25.4,17.6911045585061));
#17722=CARTESIAN_POINT('',(-25.019,6.84740300159127,-1.94289029309402E-13));
#17723=CARTESIAN_POINT('',(-17.2930919634606,6.84740300159127,18.6519919634603));
#17724=CARTESIAN_POINT('',(-25.019,25.4,-1.94289029309402E-13));
#17725=CARTESIAN_POINT('Origin',(-17.6911045585062,25.4,17.6911045585061));
#17726=CARTESIAN_POINT('',(-1.11022302462516E-12,3.7338,25.019));
#17727=CARTESIAN_POINT('',(10.1856091757486,3.7338,29.2380174616269));
#17728=CARTESIAN_POINT('',(-1.11022302462516E-12,6.84740300159127,25.019));
#17729=CARTESIAN_POINT('',(-1.11022302462516E-12,25.4,25.019));
#17730=CARTESIAN_POINT('',(14.8292874049544,6.84740300159127,31.1614919634607));
#17731=CARTESIAN_POINT('Origin',(-1.11022302462516E-12,25.4,25.019));
#17732=CARTESIAN_POINT('',(17.6911045585062,3.7338,17.691104558506));
#17733=CARTESIAN_POINT('',(27.8767137342539,3.7338,13.4720870968792));
#17734=CARTESIAN_POINT('',(17.6911045585062,6.84740300159127,17.691104558506));
#17735=CARTESIAN_POINT('',(17.6911045585062,25.4,17.691104558506));
#17736=CARTESIAN_POINT('',(32.5203919634596,6.84740300159127,11.5486125950456));
#17737=CARTESIAN_POINT('Origin',(17.6911045585062,25.4,17.691104558506));
#17738=CARTESIAN_POINT('',(25.019,3.7338,-1.11022302462516E-13));
#17739=CARTESIAN_POINT('',(24.6202833695062,3.7338,0.962587096878853));
#17740=CARTESIAN_POINT('',(25.019,6.84740300159127,-1.11022302462516E-13));
#17741=CARTESIAN_POINT('',(25.019,25.4,-1.11022302462516E-13));
#17742=CARTESIAN_POINT('',(25.4170125950456,6.84740300159127,-0.960887404954397));
#17743=CARTESIAN_POINT('Origin',(25.019,25.4,-1.11022302462516E-13));
#17744=CARTESIAN_POINT('',(17.6911045585053,3.7338,-17.6911045585064));
#17745=CARTESIAN_POINT('',(24.6202833695073,3.7338,-0.962587096879686));
#17746=CARTESIAN_POINT('',(17.6911045585053,6.84740300159127,-17.6911045585064));
#17747=CARTESIAN_POINT('',(17.6911045585053,25.4,-17.6911045585064));
#17748=CARTESIAN_POINT('',(25.4170125950445,6.84740300159127,0.960887404954397));
#17749=CARTESIAN_POINT('Origin',(17.6911045585053,25.4,-17.6911045585064));
#17750=CARTESIAN_POINT('',(0.,3.7338,-25.019));
#17751=CARTESIAN_POINT('',(27.876713734255,3.7338,-13.4720870968792));
#17752=CARTESIAN_POINT('',(0.,6.84740300159127,-25.019));
#17753=CARTESIAN_POINT('',(0.,25.4,-25.019));
#17754=CARTESIAN_POINT('',(32.5203919634607,6.84740300159127,-11.5486125950456));
#17755=CARTESIAN_POINT('Origin',(0.,25.4,-25.019));
#17756=CARTESIAN_POINT('',(-17.6911045585071,3.7338,-17.6911045585063));
#17757=CARTESIAN_POINT('',(10.1856091757476,3.7338,-29.2380174616269));
#17758=CARTESIAN_POINT('',(-17.6911045585071,6.84740300159127,-17.6911045585063));
#17759=CARTESIAN_POINT('',(-17.6911045585071,25.4,-17.6911045585063));
#17760=CARTESIAN_POINT('',(14.8292874049533,6.84740300159127,-31.1614919634607));
#17761=CARTESIAN_POINT('Origin',(-17.6911045585071,25.4,-17.6911045585063));
#17762=CARTESIAN_POINT('',(-18.089821189,3.7338,-16.7285174616273));
#17763=CARTESIAN_POINT('',(-17.2930919634617,6.84740300159127,-18.651991963461));
#17764=CARTESIAN_POINT('Origin',(27.7368,6.84740300159127,0.));
#17765=CARTESIAN_POINT('Origin',(22.2963925452559,3.7338,0.));
#17766=CARTESIAN_POINT('Origin',(5.63880000000005,0.,0.));
#17767=CARTESIAN_POINT('Origin',(8.08989999999998,3.048,-6.66133814775094E-13));
#17981=UNCERTAINTY_MEASURE_WITH_UNIT(LENGTH_MEASURE(0.01),#18007,
'DISTANCE_ACCURACY_VALUE',
'Maximum model space distance between geometric entities at asserted c
onnectivities');
#17986=UNCERTAINTY_MEASURE_WITH_UNIT(LENGTH_MEASURE(0.01),#18007,
'DISTANCE_ACCURACY_VALUE',
'Maximum model space distance between geometric entities at asserted c
onnectivities');
#18001=(
GEOMETRIC_REPRESENTATION_CONTEXT(3)
GLOBAL_UNCERTAINTY_ASSIGNED_CONTEXT((#17981))
GLOBAL_UNIT_ASSIGNED_CONTEXT((#18007,#18009,#18010))
REPRESENTATION_CONTEXT('','3D')
);
#18006=(
GEOMETRIC_REPRESENTATION_CONTEXT(3)
GLOBAL_UNCERTAINTY_ASSIGNED_CONTEXT((#17986))
GLOBAL_UNIT_ASSIGNED_CONTEXT((#18007,#18009,#18010))
REPRESENTATION_CONTEXT('','3D')
);
#18007=(
LENGTH_UNIT()
NAMED_UNIT(*)
SI_UNIT(.MILLI.,.METRE.)
);
#18009=(
NAMED_UNIT(*)
PLANE_ANGLE_UNIT()
SI_UNIT($,.RADIAN.)
);
#18010=(
NAMED_UNIT(*)
SI_UNIT($,.STERADIAN.)
SOLID_ANGLE_UNIT()
);
#18025=SHAPE_DEFINITION_REPRESENTATION(#18044,#18084);
#18044=PRODUCT_DEFINITION_SHAPE('',$,#18104);
#18084=SHAPE_REPRESENTATION('',(#10683),#18001);
#18089=PRODUCT_DEFINITION_CONTEXT('part definition',#18148,'design');
#18104=PRODUCT_DEFINITION('Caster Mounting Plate',
'Caster Mounting Plate',#18123,#18089);
#18123=PRODUCT_DEFINITION_FORMATION('',$,#18164);
#18148=APPLICATION_CONTEXT(
'Core Data for Automotive Mechanical Design Process');
#18149=PRODUCT_CONTEXT('part definition',#18148,'mechanical');
#18164=PRODUCT('Caster Mounting Plate','Caster Mounting Plate',$,(#18149));
#18172=PRESENTATION_STYLE_ASSIGNMENT((#18176));
#18176=SURFACE_STYLE_USAGE(.BOTH.,#18180);
#18180=SURFACE_SIDE_STYLE('',(#18184));
#18184=SURFACE_STYLE_FILL_AREA(#18188);
#18188=FILL_AREA_STYLE('Opaque(97,158,199)',(#18192));
#18192=FILL_AREA_STYLE_COLOUR('Opaque(97,158,199)',#18196);
#18196=COLOUR_RGB('Opaque(97,158,199)',0.380392156862745,0.619607843137255,
0.780392156862745);
ENDSEC;
END-ISO-10303-21;
